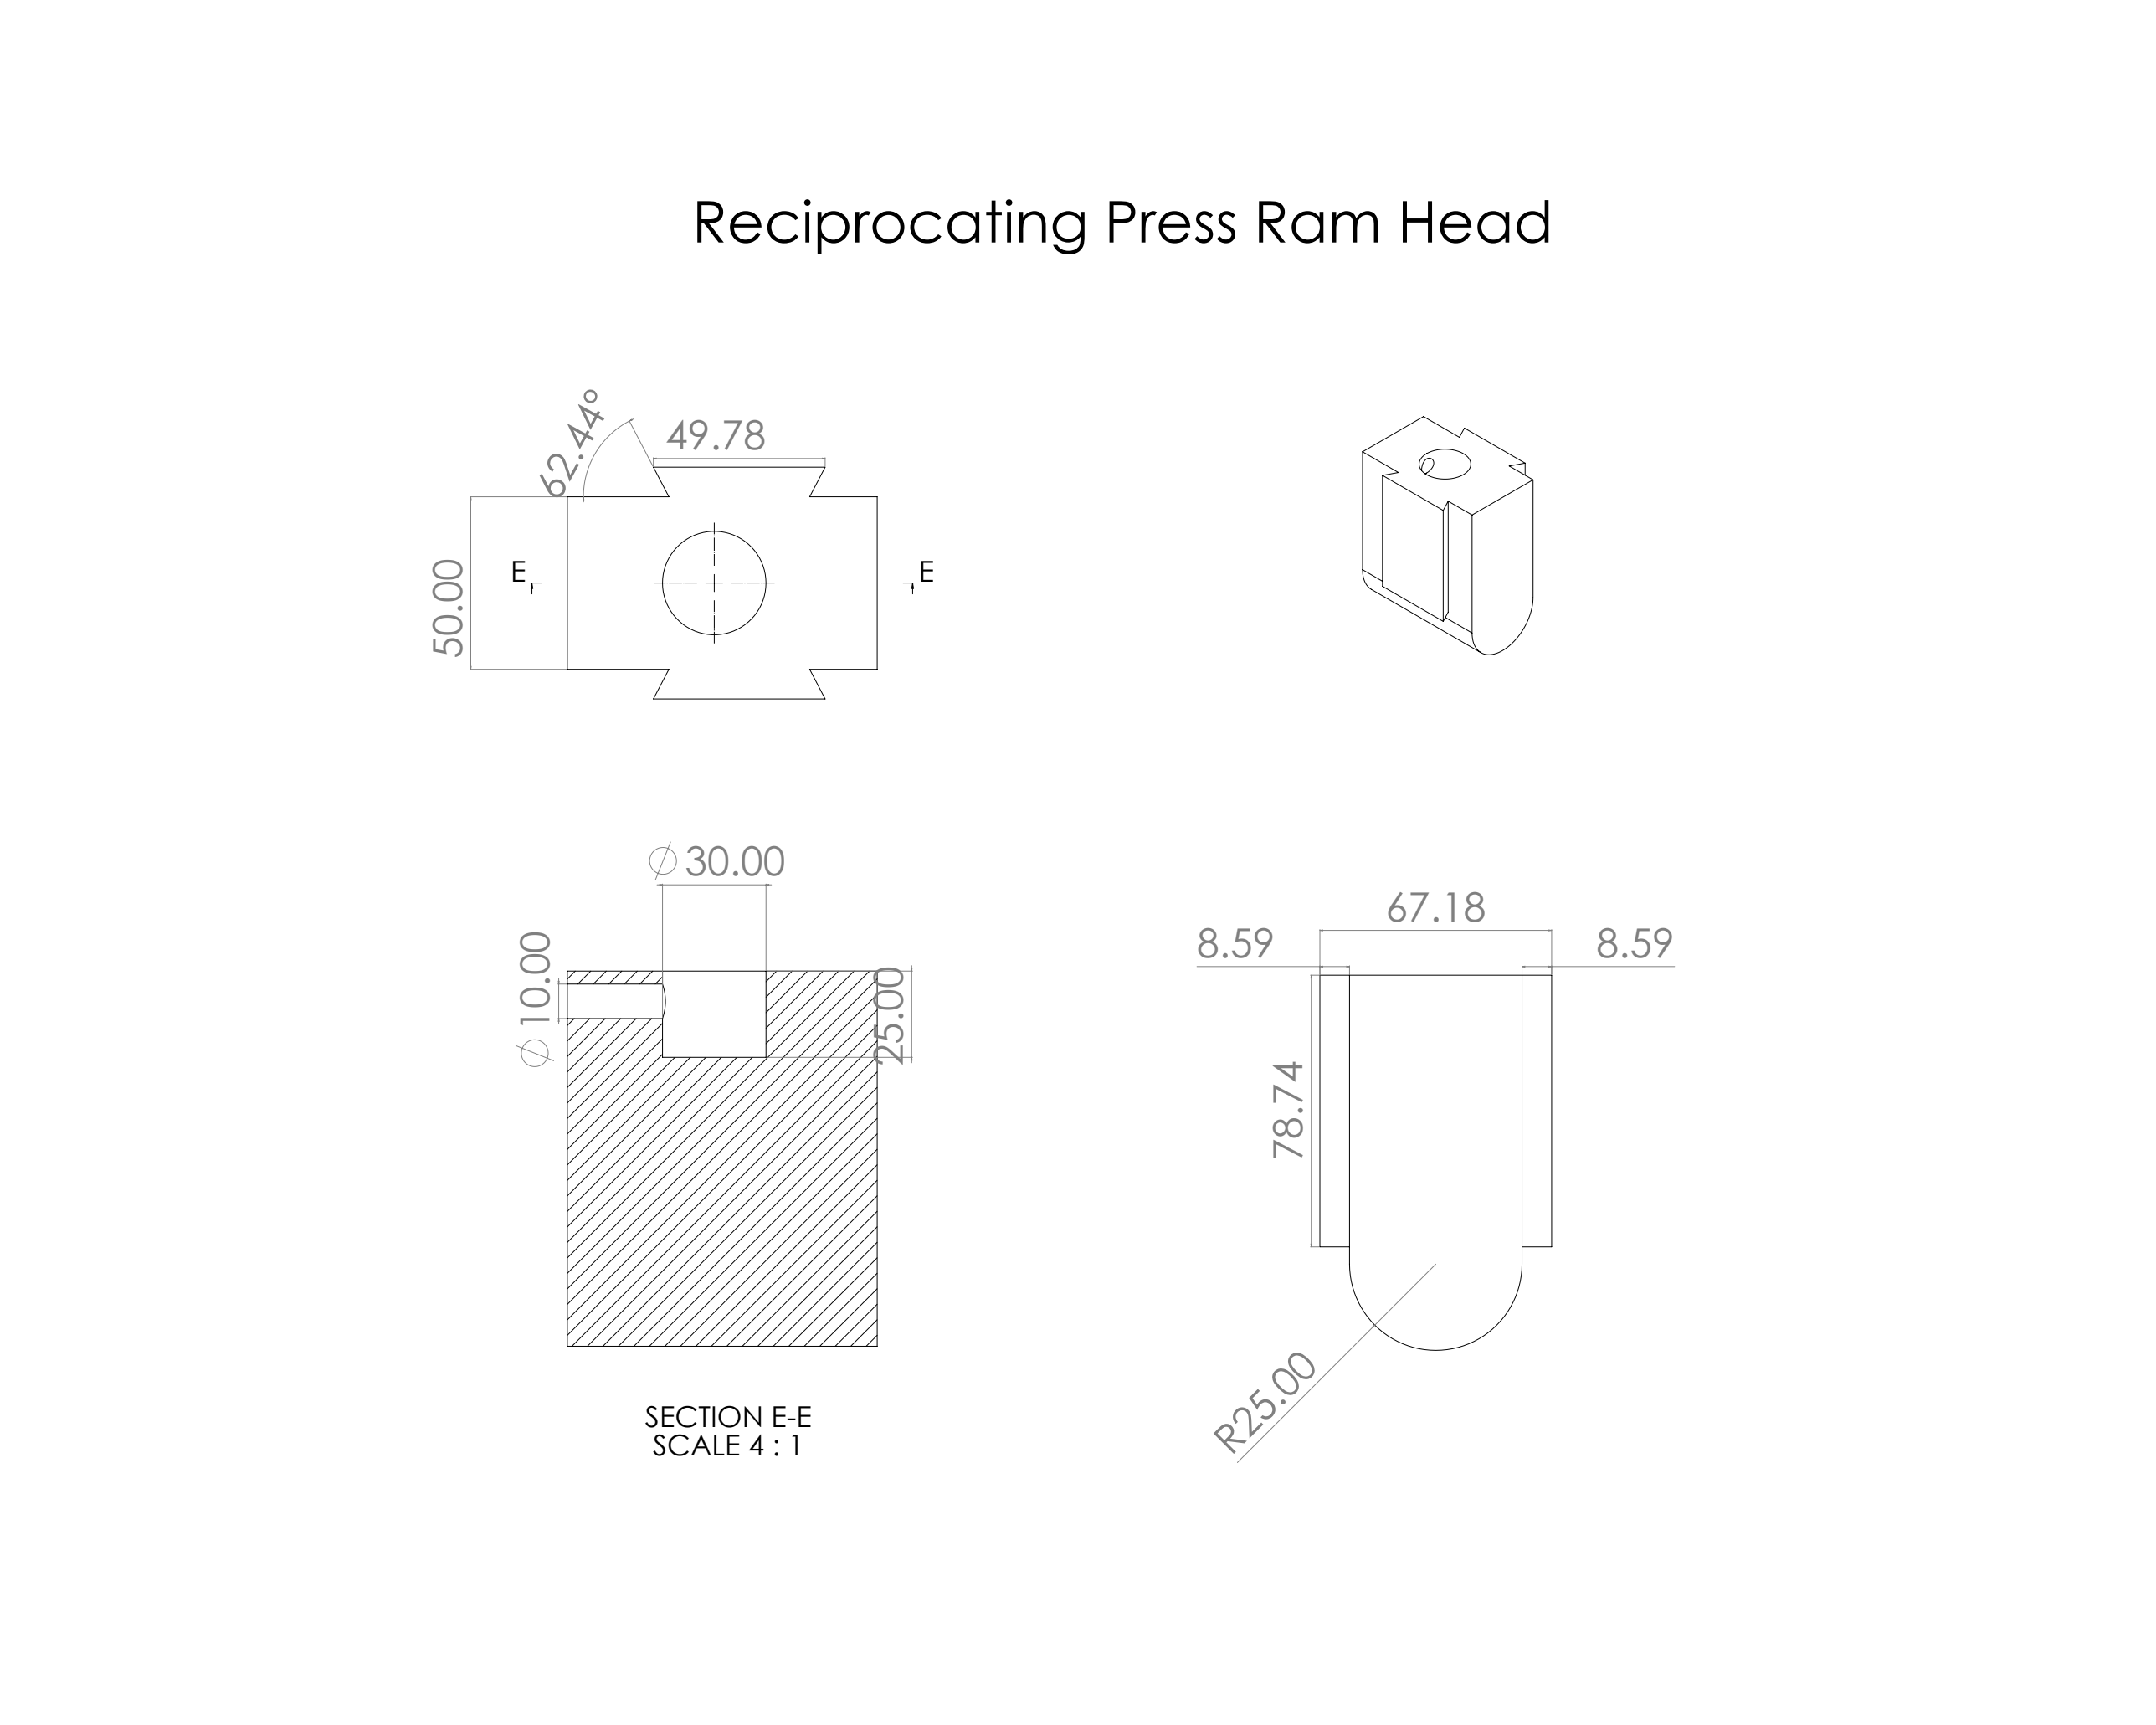
ISO-10303-21;
HEADER;
FILE_DESCRIPTION (('STEP AP214'),
    '1' );
FILE_NAME ('Reciprocating Press Ram Head.step',
    '2026-10-24T00:28:05',
    ( '' ),
    ( '' ),
    'SwSTEP 2.0',
    'SolidWorks 2025',
    '' );
FILE_SCHEMA (( 'AUTOMOTIVE_DESIGN' ));
ENDSEC;

DATA;
#14=CARTESIAN_POINT ( 'NONE',  ( -43.04716123355245827, 207.6569251493015429, -4.334626618252813479 ) ) ;
#38=EDGE_CURVE ( 'NONE', #12347, #13852, #5030, .T. ) ;
#51=CIRCLE ( 'NONE', #12122, 25.00000000000000711 ) ;
#74=VERTEX_POINT ( 'NONE', #5769 ) ;
#92=CARTESIAN_POINT ( 'NONE',  ( 3.458603197740078627, 135.1716627696692683, -33.59072564020503648 ) ) ;
#250=EDGE_CURVE ( 'NONE', #13614, #661, #3833, .T. ) ;
#262=ORIENTED_EDGE ( 'NONE', *, *, #2754, .T. ) ;
#275=CARTESIAN_POINT ( 'NONE',  ( 18.55315245287936321, 326.0737056351150613, 0.000000000000000000 ) ) ;
#276=DIRECTION ( 'NONE',  ( 1.000000000000000000, 0.000000000000000000, 0.000000000000000000 ) ) ;
#303=DIRECTION ( 'NONE',  ( 0.000000000000000000, -1.000000000000000000, 0.000000000000000000 ) ) ;
#324=PRODUCT_DEFINITION ( 'UNKNOWN', '', #14550, #16365 ) ;
#333=AXIS2_PLACEMENT_3D ( 'NONE', #2652, #9240, #18099 ) ;
#342=ORIENTED_EDGE ( 'NONE', *, *, #2095, .T. ) ;
#346=PLANE ( 'NONE',  #8685 ) ;
#375=SHAPE_DEFINITION_REPRESENTATION ( #12875, #7793 ) ;
#412=DIRECTION ( 'NONE',  ( -1.000000000000000000, 0.000000000000000000, -0.000000000000000000 ) ) ;
#463=ADVANCED_FACE ( 'NONE', ( #4898 ), #18196, .F. ) ;
#483=DIRECTION ( 'NONE',  ( 0.000000000000000000, -1.000000000000000000, 0.000000000000000000 ) ) ;
#546=ORIENTED_EDGE ( 'NONE', *, *, #13520, .F. ) ;
#560=EDGE_CURVE ( 'NONE', #9549, #9782, #17331, .T. ) ;
#593=CARTESIAN_POINT ( 'NONE',  ( -42.91927816222971614, 203.5270276421415190, -4.734255112268845878 ) ) ;
#601=VECTOR ( 'NONE', #13140, 999.9999999999998863 ) ;
#613=VECTOR ( 'NONE', #276, 1000.000000000000000 ) ;
#616=DIRECTION ( 'NONE',  ( -1.191790137725560488E-16, 1.000000000000000000, -0.000000000000000000 ) ) ;
#661=VERTEX_POINT ( 'NONE', #1116 ) ;
#674=CARTESIAN_POINT ( 'NONE',  ( -1.025382690249029949, 326.0737056351150613, 25.00000000000000000 ) ) ;
#696=DIRECTION ( 'NONE',  ( 1.000000000000000000, 0.000000000000000000, 0.000000000000000000 ) ) ;
#777=EDGE_CURVE ( 'NONE', #1912, #13157, #11419, .T. ) ;
#808=CARTESIAN_POINT ( 'NONE',  ( 0.000000000000000000, 0.000000000000000000, 0.000000000000000000 ) ) ;
#811=CARTESIAN_POINT ( 'NONE',  ( -43.67482055103364047, 200.1767183643995054, -0.6599055232175776720 ) ) ;
#849=AXIS2_PLACEMENT_3D ( 'NONE', #5042, #1929, #16634 ) ;
#854=DIRECTION ( 'NONE',  ( -1.000000000000000000, -0.000000000000000000, -0.000000000000000000 ) ) ;
#866=CARTESIAN_POINT ( 'NONE',  ( -1.025382690249028173, 213.9102039777116602, -25.00000000000000000 ) ) ;
#873=ORIENTED_EDGE ( 'NONE', *, *, #38, .F. ) ;
#897=ORIENTED_EDGE ( 'NONE', *, *, #15663, .F. ) ;
#937=FACE_OUTER_BOUND ( 'NONE', #6121, .T. ) ;
#962=DIRECTION ( 'NONE',  ( 0.000000000000000000, 0.000000000000000000, 1.000000000000000000 ) ) ;
#1045=CARTESIAN_POINT ( 'NONE',  ( -31.26501780185373391, 205.1437886375728965, 0.000000000000000000 ) ) ;
#1104=EDGE_CURVE ( 'NONE', #13157, #1912, #14909, .T. ) ;
#1113=AXIS2_PLACEMENT_3D ( 'NONE', #20332, #2170, #13424 ) ;
#1116=CARTESIAN_POINT ( 'NONE',  ( 3.458603197740078627, 213.9102039777116602, -33.59072564020503648 ) ) ;
#1153=FACE_OUTER_BOUND ( 'NONE', #10681, .T. ) ;
#1176=EDGE_CURVE ( 'NONE', #7385, #13157, #2466, .T. ) ;
#1212=ORIENTED_EDGE ( 'NONE', *, *, #6430, .T. ) ;
#1228=LINE ( 'NONE', #14432, #10712 ) ;
#1281=AXIS2_PLACEMENT_3D ( 'NONE', #20836, #19309, #9358 ) ;
#1284=EDGE_CURVE ( 'NONE', #6399, #21098, #51, .T. ) ;
#1288=ORIENTED_EDGE ( 'NONE', *, *, #5130, .F. ) ;
#1300=B_SPLINE_CURVE_WITH_KNOTS ( 'NONE', 3,
 ( #11564, #18152, #4544, #3349, #1735, #3030, #2927, #6576, #14505, #8308, #6261, #13199, #9507, #9614, #16231, #12766, #7875, #6152, #21296, #12873 ),
 .UNSPECIFIED., .F., .F.,
 ( 4, 2, 2, 2, 2, 2, 2, 2, 2, 4 ),
 ( 2.332952144782239016E-18, 0.0009844208871748760543, 0.001968841774349749506, 0.002953262661524623609, 0.003937683548699497278, 0.004922104435874371381, 0.005906525323049245484, 0.006398735766636720265, 0.006890946210224195914, 0.007875367097399143743 ),
 .UNSPECIFIED. ) ;
#1317=CARTESIAN_POINT ( 'NONE',  ( -43.15102588740141698, 208.1950015687324651, -3.974285180378252402 ) ) ;
#1370=ORIENTED_EDGE ( 'NONE', *, *, #11144, .T. ) ;
#1410=VECTOR ( 'NONE', #483, 1000.000000000000000 ) ;
#1419=CARTESIAN_POINT ( 'NONE',  ( -43.47609127650945737, 209.4774105891669933, -2.515022083182098189 ) ) ;
#1471=VERTEX_POINT ( 'NONE', #17701 ) ;
#1530=VECTOR ( 'NONE', #9051, 1000.000000000000000 ) ;
#1547=EDGE_LOOP ( 'NONE', ( #12729, #14512, #20221, #4392 ) ) ;
#1572=CARTESIAN_POINT ( 'NONE',  ( -43.15150032496258348, 208.1972798037766950, 3.972578417695639352 ) ) ;
#1670=DIRECTION ( 'NONE',  ( 0.8865057725575725689, 0.000000000000000000, 0.4627175328665443232 ) ) ;
#1703=DIRECTION ( 'NONE',  ( -1.000000000000000000, 0.000000000000000000, 0.000000000000000000 ) ) ;
#1713=CARTESIAN_POINT ( 'NONE',  ( -13.68588794268869790, 213.9102039777116602, 1.836970198721029589E-15 ) ) ;
#1731=CARTESIAN_POINT ( 'NONE',  ( -71.26501780185373036, 213.9102039777116602, 0.000000000000000000 ) ) ;
#1735=CARTESIAN_POINT ( 'NONE',  ( -43.60108677734861260, 200.4027425691367057, 1.621665263882683838 ) ) ;
#1762=CLOSED_SHELL ( 'NONE', ( #4254, #7700, #10763, #5705, #463, #10790, #10403, #16061, #9033, #19364, #19712, #8820, #7218, #3065, #7846, #20538, #4593, #3084, #19659 ) ) ;
#1775=VECTOR ( 'NONE', #9135, 1000.000000000000000 ) ;
#1776=AXIS2_PLACEMENT_3D ( 'NONE', #17630, #12444, #5836 ) ;
#1798=CARTESIAN_POINT ( 'NONE',  ( -43.47642916300955562, 209.4785612017895176, 2.513052019990858366 ) ) ;
#1846=CARTESIAN_POINT ( 'NONE',  ( 1.336753550880579347E-14, 213.9102039777116602, 25.00000000000000000 ) ) ;
#1896=CARTESIAN_POINT ( 'NONE',  ( 18.55315245287936321, 326.0737056351150613, 25.00000000000000000 ) ) ;
#1906=CARTESIAN_POINT ( 'NONE',  ( -43.68320130047528238, 210.1357463702879613, 0.3279153920022773727 ) ) ;
#1912=VERTEX_POINT ( 'NONE', #6308 ) ;
#1929=DIRECTION ( 'NONE',  ( -1.191790137725560488E-16, 1.000000000000000000, 0.000000000000000000 ) ) ;
#2094=VECTOR ( 'NONE', #11631, 1000.000000000000114 ) ;
#2095=EDGE_CURVE ( 'NONE', #11573, #6399, #18201, .T. ) ;
#2106=CARTESIAN_POINT ( 'NONE',  ( -43.31864445205426506, 201.3798797254112571, -3.307266650052995249 ) ) ;
#2121=VERTEX_POINT ( 'NONE', #8355 ) ;
#2170=DIRECTION ( 'NONE',  ( -1.000000000000000000, -0.000000000000000000, -0.000000000000000000 ) ) ;
#2193=CARTESIAN_POINT ( 'NONE',  ( -43.68588794268869435, 188.9102039777116602, 0.000000000000000000 ) ) ;
#2208=CARTESIAN_POINT ( 'NONE',  ( -43.37470026482863972, 201.1699573972600774, -3.051950158715578176 ) ) ;
#2235=PLANE ( 'NONE',  #7704 ) ;
#2269=ORIENTED_EDGE ( 'NONE', *, *, #15543, .T. ) ;
#2275=DIRECTION ( 'NONE',  ( 0.000000000000000000, 0.000000000000000000, -1.000000000000000000 ) ) ;
#2326=EDGE_LOOP ( 'NONE', ( #21282, #8318, #9603, #19499 ) ) ;
#2355=ORIENTED_EDGE ( 'NONE', *, *, #18512, .F. ) ;
#2419=DIRECTION ( 'NONE',  ( 0.000000000000000000, 0.000000000000000000, 1.000000000000000000 ) ) ;
#2422=DIRECTION ( 'NONE',  ( 0.4627175328665443232, 5.514621922230504147E-17, 0.8865057725575725689 ) ) ;
#2466=LINE ( 'NONE', #17179, #15585 ) ;
#2470=CARTESIAN_POINT ( 'NONE',  ( 1.336753550880579347E-14, 213.9102039777116602, -25.00000000000000000 ) ) ;
#2514=CARTESIAN_POINT ( 'NONE',  ( -46.31968306282883674, 326.0737056351150613, -33.59072564020502938 ) ) ;
#2554=LINE ( 'NONE', #8817, #1775 ) ;
#2611=EDGE_CURVE ( 'NONE', #18039, #6038, #13957, .T. ) ;
#2652=CARTESIAN_POINT ( 'NONE',  ( 0.000000000000000000, 326.0737056351150613, -33.59072564020503648 ) ) ;
#2754=EDGE_CURVE ( 'NONE', #10000, #13614, #15997, .T. ) ;
#2791=VECTOR ( 'NONE', #17043, 999.9999999999998863 ) ;
#2810=LINE ( 'NONE', #19027, #18368 ) ;
#2818=CARTESIAN_POINT ( 'NONE',  ( -71.26501780185373036, 135.1716627696692683, -25.00000000000000000 ) ) ;
#2841=DIRECTION ( 'NONE',  ( 1.191790137725560488E-16, -1.000000000000000000, 0.000000000000000000 ) ) ;
#2860=FACE_OUTER_BOUND ( 'NONE', #2326, .T. ) ;
#2875=DIRECTION ( 'NONE',  ( -1.000000000000000000, 0.000000000000000000, 0.000000000000000000 ) ) ;
#2885=EDGE_LOOP ( 'NONE', ( #4892, #17666 ) ) ;
#2927=CARTESIAN_POINT ( 'NONE',  ( -43.47648769733579854, 200.8087914445877971, 2.512805286998617049 ) ) ;
#2965=DIRECTION ( 'NONE',  ( -0.8865057725575725689, 0.000000000000000000, 0.4627175328665443232 ) ) ;
#2978=FACE_OUTER_BOUND ( 'NONE', #14370, .T. ) ;
#2988=ORIENTED_EDGE ( 'NONE', *, *, #21108, .T. ) ;
#3004=DIRECTION ( 'NONE',  ( 0.000000000000000000, 0.000000000000000000, 1.000000000000000000 ) ) ;
#3030=CARTESIAN_POINT ( 'NONE',  ( -43.52287249567941529, 200.6548609068916278, 2.226397062484288814 ) ) ;
#3065=ADVANCED_FACE ( 'NONE', ( #16524, #8276 ), #13386, .T. ) ;
#3066=AXIS2_PLACEMENT_3D ( 'NONE', #16187, #11087, #4703 ) ;
#3084=ADVANCED_FACE ( 'NONE', ( #13280 ), #3533, .T. ) ;
#3104=CARTESIAN_POINT ( 'NONE',  ( -28.68588794268869435, 188.9102039777116602, 0.000000000000000000 ) ) ;
#3152=VECTOR ( 'NONE', #5219, 1000.000000000000000 ) ;
#3194=CARTESIAN_POINT ( 'NONE',  ( -43.04742826731176564, 207.6584868706943041, 4.333760535973598671 ) ) ;
#3226=VECTOR ( 'NONE', #10704, 1000.000000000000000 ) ;
#3249=ORIENTED_EDGE ( 'NONE', *, *, #10862, .T. ) ;
#3255=CARTESIAN_POINT ( 'NONE',  ( -43.31915179403467420, 208.9097650327693430, -3.305147470758842410 ) ) ;
#3297=DIRECTION ( 'NONE',  ( 0.8865057725575725689, 0.000000000000000000, 0.4627175328665443232 ) ) ;
#3308=ORIENTED_EDGE ( 'NONE', *, *, #21108, .F. ) ;
#3314=ORIENTED_EDGE ( 'NONE', *, *, #18512, .T. ) ;
#3321=DIRECTION ( 'NONE',  ( 0.000000000000000000, -0.000000000000000000, -1.000000000000000000 ) ) ;
#3332=VECTOR ( 'NONE', #8114, 1000.000000000000000 ) ;
#3349=CARTESIAN_POINT ( 'NONE',  ( -43.63268616469407846, 200.3053519615658615, 1.302651870180923321 ) ) ;
#3359=VERTEX_POINT ( 'NONE', #2193 ) ;
#3397=DIRECTION ( 'NONE',  ( 0.000000000000000000, -1.000000000000000000, 0.000000000000000000 ) ) ;
#3415=ORIENTED_EDGE ( 'NONE', *, *, #8284, .T. ) ;
#3448=CARTESIAN_POINT ( 'NONE',  ( -41.83569717483972994, 135.1716627696692683, -24.99999999999998934 ) ) ;
#3488=( GEOMETRIC_REPRESENTATION_CONTEXT ( 3 ) GLOBAL_UNCERTAINTY_ASSIGNED_CONTEXT ( ( #13089 ) ) GLOBAL_UNIT_ASSIGNED_CONTEXT ( ( #13667, #8565, #20256 ) ) REPRESENTATION_CONTEXT ( 'NONE', 'WORKASPACE' ) );
#3507=CARTESIAN_POINT ( 'NONE',  ( -22.62331590640576096, 213.9102039777116602, -11.80838889663596447 ) ) ;
#3524=AXIS2_PLACEMENT_3D ( 'NONE', #11422, #7749, #3004 ) ;
#3533=PLANE ( 'NONE',  #849 ) ;
#3542=EDGE_CURVE ( 'NONE', #16754, #11704, #13661, .T. ) ;
#3567=VERTEX_POINT ( 'NONE', #5738 ) ;
#3679=ORIENTED_EDGE ( 'NONE', *, *, #2611, .T. ) ;
#3786=EDGE_CURVE ( 'NONE', #15417, #3359, #12531, .T. ) ;
#3794=ORIENTED_EDGE ( 'NONE', *, *, #5782, .T. ) ;
#3830=DIRECTION ( 'NONE',  ( -0.8865057725575725689, 0.000000000000000000, 0.4627175328665443232 ) ) ;
#3833=LINE ( 'NONE', #7069, #2791 ) ;
#3840=VECTOR ( 'NONE', #2422, 999.9999999999998863 ) ;
#3876=CARTESIAN_POINT ( 'NONE',  ( -22.62331590640576451, 135.1716627696692683, -11.80838889663595914 ) ) ;
#3922=EDGE_CURVE ( 'NONE', #14679, #13370, #6472, .T. ) ;
#3937=CARTESIAN_POINT ( 'NONE',  ( -43.68588794268869435, 200.1437886375728965, 2.403080215999224424E-15 ) ) ;
#3952=DIRECTION ( 'NONE',  ( -1.000000000000000000, -1.191790137725560488E-16, 0.000000000000000000 ) ) ;
#3982=ORIENTED_EDGE ( 'NONE', *, *, #15019, .F. ) ;
#3983=ORIENTED_EDGE ( 'NONE', *, *, #17042, .T. ) ;
#4031=CARTESIAN_POINT ( 'NONE',  ( -22.62331590640576096, 213.9102039777116602, 11.80838889663596447 ) ) ;
#4043=FACE_OUTER_BOUND ( 'NONE', #8124, .T. ) ;
#4177=EDGE_LOOP ( 'NONE', ( #3308, #13446, #6905, #1212 ) ) ;
#4245=AXIS2_PLACEMENT_3D ( 'NONE', #13600, #303, #3321 ) ;
#4254=ADVANCED_FACE ( 'NONE', ( #6341 ), #7319, .F. ) ;
#4312=DIRECTION ( 'NONE',  ( -0.4627175328665442677, 0.000000000000000000, 0.8865057725575725689 ) ) ;
#4315=CARTESIAN_POINT ( 'NONE',  ( -1.025382690249029949, 213.9102039777116602, 25.00000000000000000 ) ) ;
#4335=EDGE_CURVE ( 'NONE', #6728, #10701, #7955, .T. ) ;
#4342=ORIENTED_EDGE ( 'NONE', *, *, #777, .T. ) ;
#4379=DIRECTION ( 'NONE',  ( 0.000000000000000000, -1.000000000000000000, 0.000000000000000000 ) ) ;
#4387=AXIS2_PLACEMENT_3D ( 'NONE', #9664, #8472, #8251 ) ;
#4392=ORIENTED_EDGE ( 'NONE', *, *, #1284, .F. ) ;
#4443=ORIENTED_EDGE ( 'NONE', *, *, #4335, .T. ) ;
#4447=PLANE ( 'NONE',  #8269 ) ;
#4449=DIRECTION ( 'NONE',  ( 0.000000000000000000, 0.000000000000000000, 1.000000000000000000 ) ) ;
#4452=FACE_BOUND ( 'NONE', #15353, .T. ) ;
#4489=LINE ( 'NONE', #12925, #9062 ) ;
#4544=CARTESIAN_POINT ( 'NONE',  ( -43.67481775055303928, 200.1767262095909246, 0.6600471188826699809 ) ) ;
#4553=CARTESIAN_POINT ( 'NONE',  ( -42.91697296918459159, 206.7606908932681051, -4.742769269235594720 ) ) ;
#4593=ADVANCED_FACE ( 'NONE', ( #1153 ), #16179, .F. ) ;
#4613=CARTESIAN_POINT ( 'NONE',  ( -13.68588794268869435, 188.9102039777116602, 1.836970198721029983E-15 ) ) ;
#4646=LINE ( 'NONE', #16443, #16857 ) ;
#4663=DIRECTION ( 'NONE',  ( 1.000000000000000000, 1.191790137725560488E-16, 0.000000000000000000 ) ) ;
#4691=CARTESIAN_POINT ( 'NONE',  ( -71.26501780185373036, 130.1716627696692683, 25.00000000000000000 ) ) ;
#4703=DIRECTION ( 'NONE',  ( -1.000000000000000000, 0.000000000000000000, 0.000000000000000000 ) ) ;
#4757=CARTESIAN_POINT ( 'NONE',  ( -42.88446638378037079, 206.4484180351192322, -4.837872587287148640 ) ) ;
#4764=CARTESIAN_POINT ( 'NONE',  ( -28.68588794268869790, 213.9102039777116602, 0.000000000000000000 ) ) ;
#4773=CARTESIAN_POINT ( 'NONE',  ( -42.82802356641964536, 205.1437886375728965, -5.000000000000001776 ) ) ;
#4892=ORIENTED_EDGE ( 'NONE', *, *, #1104, .F. ) ;
#4898=FACE_OUTER_BOUND ( 'NONE', #12108, .T. ) ;
#4920=VERTEX_POINT ( 'NONE', #20370 ) ;
#4926=EDGE_CURVE ( 'NONE', #13370, #10360, #12699, .T. ) ;
#4933=DIRECTION ( 'NONE',  ( -1.191790137725560488E-16, 1.000000000000000000, 0.000000000000000000 ) ) ;
#4946=VECTOR ( 'NONE', #13315, 1000.000000000000000 ) ;
#4962=LINE ( 'NONE', #2818, #8189 ) ;
#4973=ORIENTED_EDGE ( 'NONE', *, *, #2754, .F. ) ;
#5019=CARTESIAN_POINT ( 'NONE',  ( -43.37443857369948574, 209.1166545091122657, 3.053198389463522844 ) ) ;
#5021=CARTESIAN_POINT ( 'NONE',  ( 1.336753550880579347E-14, 213.9102039777116602, 33.59072564020503648 ) ) ;
#5030=LINE ( 'NONE', #18331, #2094 ) ;
#5033=ORIENTED_EDGE ( 'NONE', *, *, #4335, .F. ) ;
#5042=CARTESIAN_POINT ( 'NONE',  ( -28.68588794268869435, 188.9102039777116602, 0.000000000000000000 ) ) ;
#5077=EDGE_CURVE ( 'NONE', #9549, #20916, #15731, .T. ) ;
#5120=FACE_OUTER_BOUND ( 'NONE', #14147, .T. ) ;
#5130=EDGE_CURVE ( 'NONE', #1471, #2121, #1228, .T. ) ;
#5135=AXIS2_PLACEMENT_3D ( 'NONE', #4764, #2841, #4663 ) ;
#5215=ORIENTED_EDGE ( 'NONE', *, *, #250, .T. ) ;
#5219=DIRECTION ( 'NONE',  ( 0.000000000000000000, -1.000000000000000000, 0.000000000000000000 ) ) ;
#5265=ORIENTED_EDGE ( 'NONE', *, *, #5077, .T. ) ;
#5460=CARTESIAN_POINT ( 'NONE',  ( 1.631480618821192334E-14, 213.9102039777116602, -24.99999999999999645 ) ) ;
#5464=LINE ( 'NONE', #1731, #10962 ) ;
#5507=ORIENTED_EDGE ( 'NONE', *, *, #20586, .F. ) ;
#5529=DIRECTION ( 'NONE',  ( -0.4627175328665442677, 0.000000000000000000, -0.8865057725575725689 ) ) ;
#5616=ORIENTED_EDGE ( 'NONE', *, *, #5775, .F. ) ;
#5629=ORIENTED_EDGE ( 'NONE', *, *, #2095, .F. ) ;
#5634=LINE ( 'NONE', #17220, #3226 ) ;
#5675=DIRECTION ( 'NONE',  ( 1.000000000000000000, 1.191790137725560488E-16, 1.178908271762451515E-16 ) ) ;
#5677=CARTESIAN_POINT ( 'NONE',  ( -41.83569717483972994, 213.9102039777116602, -25.00000000000000000 ) ) ;
#5705=ADVANCED_FACE ( 'NONE', ( #10914 ), #17526, .T. ) ;
#5738=CARTESIAN_POINT ( 'NONE',  ( -43.68588794268869435, 213.9102039777116602, 0.000000000000000000 ) ) ;
#5769=CARTESIAN_POINT ( 'NONE',  ( -71.26501780185373036, 213.9102039777116602, 25.00000000000000355 ) ) ;
#5775=EDGE_CURVE ( 'NONE', #18006, #3567, #13504, .T. ) ;
#5782=EDGE_CURVE ( 'NONE', #10000, #11573, #19357, .T. ) ;
#5836=DIRECTION ( 'NONE',  ( -1.000000000000000000, 0.000000000000000000, 0.000000000000000000 ) ) ;
#5848=ORIENTED_EDGE ( 'NONE', *, *, #1176, .T. ) ;
#5866=CARTESIAN_POINT ( 'NONE',  ( -42.88696169552118675, 203.8418613323790396, -4.830328443944832628 ) ) ;
#5969=( NAMED_UNIT ( * ) PLANE_ANGLE_UNIT ( ) SI_UNIT ( $, .RADIAN. ) );
#6018=ORIENTED_EDGE ( 'NONE', *, *, #12630, .T. ) ;
#6038=VERTEX_POINT ( 'NONE', #11054 ) ;
#6055=ORIENTED_EDGE ( 'NONE', *, *, #560, .F. ) ;
#6121=EDGE_LOOP ( 'NONE', ( #15052, #21157, #12224, #6055 ) ) ;
#6149=CARTESIAN_POINT ( 'NONE',  ( 18.55315245287936321, 213.9102039777116602, -25.00000000000000000 ) ) ;
#6152=CARTESIAN_POINT ( 'NONE',  ( -42.83951137863823533, 204.4886979175576016, 4.967857365464206865 ) ) ;
#6261=CARTESIAN_POINT ( 'NONE',  ( -43.15146482487497792, 202.0901544311013538, 3.972812079771462113 ) ) ;
#6301=EDGE_CURVE ( 'NONE', #74, #4920, #5634, .T. ) ;
#6308=CARTESIAN_POINT ( 'NONE',  ( -71.26501780185373036, 205.1437886375728965, -5.000000000000001776 ) ) ;
#6341=FACE_OUTER_BOUND ( 'NONE', #20011, .T. ) ;
#6375=CARTESIAN_POINT ( 'NONE',  ( -43.63240530816146645, 209.9813655751484305, -1.306613905557860500 ) ) ;
#6399=VERTEX_POINT ( 'NONE', #16452 ) ;
#6430=EDGE_CURVE ( 'NONE', #6038, #16754, #8207, .T. ) ;
#6445=EDGE_CURVE ( 'NONE', #2121, #4920, #17049, .T. ) ;
#6472=B_SPLINE_CURVE_WITH_KNOTS ( 'NONE', 3,
 ( #16134, #21099, #16243, #6375, #11247, #17845, #1419, #14837, #3255, #6480, #1317, #14, #19576, #4553, #4757, #6588, #11574, #7888 ),
 .UNSPECIFIED., .F., .F.,
 ( 4, 2, 2, 2, 2, 2, 2, 2, 4 ),
 ( 0.01574578602456870244, 0.01672957298347709995, 0.01771335994238549399, 0.01869714690129389151, 0.01968093386020228555, 0.02066472081911068306, 0.02164850777801907711, 0.02263229473692747462, 0.02361608169583586866 ),
 .UNSPECIFIED. ) ;
#6480=CARTESIAN_POINT ( 'NONE',  ( -43.20717515250593266, 208.4480206960199382, -3.766779594902115225 ) ) ;
#6497=LINE ( 'NONE', #14958, #11620 ) ;
#6512=DIRECTION ( 'NONE',  ( 0.4627175328665442677, 0.000000000000000000, -0.8865057725575724579 ) ) ;
#6522=LINE ( 'NONE', #3507, #601 ) ;
#6537=ORIENTED_EDGE ( 'NONE', *, *, #6301, .T. ) ;
#6555=LINE ( 'NONE', #13175, #21295 ) ;
#6576=CARTESIAN_POINT ( 'NONE',  ( -43.37414277151795261, 201.1719893629813498, 3.054701555947804792 ) ) ;
#6588=CARTESIAN_POINT ( 'NONE',  ( -42.83993802355417557, 205.8067832142903910, -4.966639429937480088 ) ) ;
#6599=DIRECTION ( 'NONE',  ( -1.191790137725560488E-16, 1.000000000000000000, -0.000000000000000000 ) ) ;
#6634=CARTESIAN_POINT ( 'NONE',  ( -42.88454851406326185, 206.4494888775581103, 4.837634058829628714 ) ) ;
#6726=ORIENTED_EDGE ( 'NONE', *, *, #17290, .T. ) ;
#6728=VERTEX_POINT ( 'NONE', #4315 ) ;
#6745=CARTESIAN_POINT ( 'NONE',  ( -42.82802356641963826, 205.4725094246604442, 5.000000000000000888 ) ) ;
#6755=ORIENTED_EDGE ( 'NONE', *, *, #15009, .T. ) ;
#6783=ORIENTED_EDGE ( 'NONE', *, *, #12630, .F. ) ;
#6835=LINE ( 'NONE', #20042, #3152 ) ;
#6850=CARTESIAN_POINT ( 'NONE',  ( -43.68588794268869435, 210.1437886375728965, -2.161864096862809871E-19 ) ) ;
#6903=EDGE_LOOP ( 'NONE', ( #8636, #14114, #13505, #19365, #10872, #20519, #6907 ) ) ;
#6905=ORIENTED_EDGE ( 'NONE', *, *, #15663, .T. ) ;
#6907=ORIENTED_EDGE ( 'NONE', *, *, #15009, .F. ) ;
#6963=ORIENTED_EDGE ( 'NONE', *, *, #15543, .F. ) ;
#6967=ORIENTED_EDGE ( 'NONE', *, *, #15708, .T. ) ;
#7012=EDGE_LOOP ( 'NONE', ( #17895, #9415, #8615, #20147 ) ) ;
#7058=CARTESIAN_POINT ( 'NONE',  ( -42.83955070047272073, 204.4880047785818533, -4.967744786903342202 ) ) ;
#7069=CARTESIAN_POINT ( 'NONE',  ( -11.06088464903279878, 213.9102039777116602, -5.773301668816275267 ) ) ;
#7080=LINE ( 'NONE', #7184, #9238 ) ;
#7160=CARTESIAN_POINT ( 'NONE',  ( -43.52298375438361688, 200.6544955639567434, -2.225641045960684128 ) ) ;
#7180=CARTESIAN_POINT ( 'NONE',  ( -43.68588794268869435, 188.9102039777116602, 0.000000000000000000 ) ) ;
#7184=CARTESIAN_POINT ( 'NONE',  ( -46.31968306282883674, 326.0737056351150613, 33.59072564020503648 ) ) ;
#7195=ORIENTED_EDGE ( 'NONE', *, *, #3786, .T. ) ;
#7201=ORIENTED_EDGE ( 'NONE', *, *, #1104, .T. ) ;
#7218=ADVANCED_FACE ( 'NONE', ( #2860 ), #17667, .T. ) ;
#7286=VERTEX_POINT ( 'NONE', #11058 ) ;
#7319=CYLINDRICAL_SURFACE ( 'NONE', #3524, 5.000000000000001776 ) ;
#7336=ORIENTED_EDGE ( 'NONE', *, *, #3542, .T. ) ;
#7350=ORIENTED_EDGE ( 'NONE', *, *, #7856, .F. ) ;
#7385=VERTEX_POINT ( 'NONE', #12073 ) ;
#7461=ORIENTED_EDGE ( 'NONE', *, *, #16181, .F. ) ;
#7544=CIRCLE ( 'NONE', #8583, 15.00000000000000355 ) ;
#7700=ADVANCED_FACE ( 'NONE', ( #19524 ), #13149, .F. ) ;
#7701=AXIS2_PLACEMENT_3D ( 'NONE', #20118, #18058, #11680 ) ;
#7704=AXIS2_PLACEMENT_3D ( 'NONE', #11854, #18551, #412 ) ;
#7749=DIRECTION ( 'NONE',  ( -1.000000000000000000, -0.000000000000000000, -0.000000000000000000 ) ) ;
#7774=CARTESIAN_POINT ( 'NONE',  ( -41.83569717483972994, 326.0737056351150613, 24.99999999999998934 ) ) ;
#7793=SHAPE_REPRESENTATION ( 'Reciprocating Press Ram Head', ( #12794 ), #14195 ) ;
#7795=LINE ( 'NONE', #20478, #18265 ) ;
#7846=ADVANCED_FACE ( 'NONE', ( #4452, #16461 ), #19689, .F. ) ;
#7856=EDGE_CURVE ( 'NONE', #11704, #18039, #8000, .T. ) ;
#7875=CARTESIAN_POINT ( 'NONE',  ( -42.87299489053027912, 204.0036020648173292, 4.871053504435129078 ) ) ;
#7888=CARTESIAN_POINT ( 'NONE',  ( -42.82802356641964536, 205.1437886375728965, -5.000000000000001776 ) ) ;
#7890=LINE ( 'NONE', #20279, #13820 ) ;
#7899=ADVANCED_BREP_SHAPE_REPRESENTATION ( '', ( #12161, #12794 ), #14195 ) ;
#7955=LINE ( 'NONE', #21170, #17343 ) ;
#8000=LINE ( 'NONE', #17956, #20325 ) ;
#8006=CARTESIAN_POINT ( 'NONE',  ( 3.458603197740078627, 135.1716627696692683, 33.59072564020503648 ) ) ;
#8047=ORIENTED_EDGE ( 'NONE', *, *, #14360, .F. ) ;
#8114=DIRECTION ( 'NONE',  ( 0.000000000000000000, -1.000000000000000000, 0.000000000000000000 ) ) ;
#8124=EDGE_LOOP ( 'NONE', ( #2355, #4443, #2988, #7336 ) ) ;
#8151=ORIENTED_EDGE ( 'NONE', *, *, #15576, .T. ) ;
#8189=VECTOR ( 'NONE', #9402, 1000.000000000000000 ) ;
#8207=LINE ( 'NONE', #9938, #4946 ) ;
#8251=DIRECTION ( 'NONE',  ( -1.000000000000000000, 0.000000000000000000, -0.000000000000000000 ) ) ;
#8269=AXIS2_PLACEMENT_3D ( 'NONE', #11032, #3830, #10419 ) ;
#8274=DIRECTION ( 'NONE',  ( 1.000000000000000000, 1.191790137725560488E-16, -1.178908271762451515E-16 ) ) ;
#8276=FACE_OUTER_BOUND ( 'NONE', #7012, .T. ) ;
#8284=EDGE_CURVE ( 'NONE', #3359, #15417, #7544, .T. ) ;
#8308=CARTESIAN_POINT ( 'NONE',  ( -43.20715004130836689, 201.8397834041948613, 3.766744768033092328 ) ) ;
#8318=ORIENTED_EDGE ( 'NONE', *, *, #560, .T. ) ;
#8355=CARTESIAN_POINT ( 'NONE',  ( -71.26501780185373036, 130.1716627696692683, -25.00000000000000355 ) ) ;
#8389=CARTESIAN_POINT ( 'NONE',  ( -71.26501780185373036, 326.0737056351150613, 0.000000000000000000 ) ) ;
#8472=DIRECTION ( 'NONE',  ( 0.000000000000000000, 0.000000000000000000, -1.000000000000000000 ) ) ;
#8474=CARTESIAN_POINT ( 'NONE',  ( -43.67243589781770652, 210.1033101532991338, 0.6559853996653204344 ) ) ;
#8536=CYLINDRICAL_SURFACE ( 'NONE', #1113, 25.00000000000000711 ) ;
#8565=( NAMED_UNIT ( * ) PLANE_ANGLE_UNIT ( ) SI_UNIT ( $, .RADIAN. ) );
#8583=AXIS2_PLACEMENT_3D ( 'NONE', #3104, #4933, #1703 ) ;
#8615=ORIENTED_EDGE ( 'NONE', *, *, #6301, .F. ) ;
#8636=ORIENTED_EDGE ( 'NONE', *, *, #3786, .F. ) ;
#8685=AXIS2_PLACEMENT_3D ( 'NONE', #18488, #2275, #15374 ) ;
#8709=CARTESIAN_POINT ( 'NONE',  ( 1.631480618821192334E-14, 213.9102039777116602, 24.99999999999999645 ) ) ;
#8817=CARTESIAN_POINT ( 'NONE',  ( -31.26501780185373391, 205.1437886375728965, -5.000000000000001776 ) ) ;
#8820=ADVANCED_FACE ( 'NONE', ( #937 ), #17463, .T. ) ;
#8828=ORIENTED_EDGE ( 'NONE', *, *, #1176, .F. ) ;
#8860=CIRCLE ( 'NONE', #1281, 15.00000000000000000 ) ;
#8870=LINE ( 'NONE', #674, #11493 ) ;
#8918=FACE_OUTER_BOUND ( 'NONE', #11911, .T. ) ;
#8938=DIRECTION ( 'NONE',  ( -1.000000000000000000, 0.000000000000000000, 0.000000000000000000 ) ) ;
#8975=UNCERTAINTY_MEASURE_WITH_UNIT (LENGTH_MEASURE( 1.000000000000000082E-05 ), #15936, 'distance_accuracy_value', 'NONE');
#9033=ADVANCED_FACE ( 'NONE', ( #5120 ), #10192, .F. ) ;
#9043=CARTESIAN_POINT ( 'NONE',  ( 18.55315245287936321, 213.9102039777116602, 25.00000000000000000 ) ) ;
#9051=DIRECTION ( 'NONE',  ( -1.000000000000000000, -1.191790137725560488E-16, 0.000000000000000000 ) ) ;
#9062=VECTOR ( 'NONE', #4379, 1000.000000000000000 ) ;
#9109=CARTESIAN_POINT ( 'NONE',  ( -43.20748696942038691, 201.8382954020869420, -3.765466433758053011 ) ) ;
#9135=DIRECTION ( 'NONE',  ( -1.000000000000000000, -0.000000000000000000, -0.000000000000000000 ) ) ;
#9197=DIRECTION ( 'NONE',  ( -1.000000000000000000, 0.000000000000000000, 0.000000000000000000 ) ) ;
#9218=VECTOR ( 'NONE', #616, 1000.000000000000000 ) ;
#9238=VECTOR ( 'NONE', #13807, 1000.000000000000000 ) ;
#9240=DIRECTION ( 'NONE',  ( 0.000000000000000000, 0.000000000000000000, -1.000000000000000000 ) ) ;
#9297=CARTESIAN_POINT ( 'NONE',  ( 18.55315245287936321, 213.9102039777116602, 0.000000000000000000 ) ) ;
#9348=EDGE_CURVE ( 'NONE', #14679, #3567, #7795, .T. ) ;
#9358=DIRECTION ( 'NONE',  ( -1.000000000000000000, 0.000000000000000000, 0.000000000000000000 ) ) ;
#9395=ORIENTED_EDGE ( 'NONE', *, *, #11250, .T. ) ;
#9398=AXIS2_PLACEMENT_3D ( 'NONE', #10969, #11394, #2875 ) ;
#9402=DIRECTION ( 'NONE',  ( 1.000000000000000000, 0.000000000000000000, 0.000000000000000000 ) ) ;
#9415=ORIENTED_EDGE ( 'NONE', *, *, #6445, .T. ) ;
#9507=CARTESIAN_POINT ( 'NONE',  ( -42.99819559747531628, 202.9232509211816478, 4.491669896562675568 ) ) ;
#9512=ORIENTED_EDGE ( 'NONE', *, *, #20586, .T. ) ;
#9549=VERTEX_POINT ( 'NONE', #12897 ) ;
#9583=PRODUCT ( 'Reciprocating Press Ram Head', 'Reciprocating Press Ram Head', '', ( #18416 ) ) ;
#9603=ORIENTED_EDGE ( 'NONE', *, *, #10862, .F. ) ;
#9614=CARTESIAN_POINT ( 'NONE',  ( -42.93756312153262655, 203.3739285472156268, 4.679109617540635924 ) ) ;
#9664=CARTESIAN_POINT ( 'NONE',  ( 0.000000000000000000, 326.0737056351150613, 25.00000000000000000 ) ) ;
#9681=ORIENTED_EDGE ( 'NONE', *, *, #17363, .F. ) ;
#9735=DIRECTION ( 'NONE',  ( -1.000000000000000000, -0.000000000000000000, -0.000000000000000000 ) ) ;
#9782=VERTEX_POINT ( 'NONE', #16997 ) ;
#9861=CARTESIAN_POINT ( 'NONE',  ( -22.62331590640576451, 326.0737056351150613, -11.80838889663595914 ) ) ;
#9901=FACE_OUTER_BOUND ( 'NONE', #10791, .T. ) ;
#9938=CARTESIAN_POINT ( 'NONE',  ( 0.000000000000000000, 135.1716627696692683, 33.59072564020503648 ) ) ;
#9967=VECTOR ( 'NONE', #3397, 1000.000000000000000 ) ;
#9985=CARTESIAN_POINT ( 'NONE',  ( -42.99906419454241302, 207.3703986995724335, 4.488953568700488006 ) ) ;
#10000=VERTEX_POINT ( 'NONE', #6149 ) ;
#10095=CARTESIAN_POINT ( 'NONE',  ( -43.63240380007613339, 209.9813597091836641, 1.306460585600322188 ) ) ;
#10127=DIRECTION ( 'NONE',  ( 1.000000000000000000, 0.000000000000000000, 0.000000000000000000 ) ) ;
#10192=PLANE ( 'NONE',  #18959 ) ;
#10281=VERTEX_POINT ( 'NONE', #3448 ) ;
#10300=CARTESIAN_POINT ( 'NONE',  ( -43.04679578547634122, 202.6324317550694616, -4.335932898175371975 ) ) ;
#10340=CARTESIAN_POINT ( 'NONE',  ( 0.000000000000000000, 130.1716627696692683, -25.00000000000000000 ) ) ;
#10358=EDGE_LOOP ( 'NONE', ( #3415, #7195 ) ) ;
#10360=VERTEX_POINT ( 'NONE', #3937 ) ;
#10382=DIRECTION ( 'NONE',  ( 0.000000000000000000, -1.000000000000000000, 0.000000000000000000 ) ) ;
#10403=ADVANCED_FACE ( 'NONE', ( #4043 ), #4447, .F. ) ;
#10409=CARTESIAN_POINT ( 'NONE',  ( -42.93765923600280843, 203.3731313234725917, -4.678819197459183954 ) ) ;
#10419=DIRECTION ( 'NONE',  ( 0.4627175328665442677, 0.000000000000000000, 0.8865057725575724579 ) ) ;
#10452=VERTEX_POINT ( 'NONE', #16136 ) ;
#10463=EDGE_CURVE ( 'NONE', #661, #9549, #7890, .T. ) ;
#10479=VECTOR ( 'NONE', #4312, 1000.000000000000114 ) ;
#10545=B_SPLINE_CURVE_WITH_KNOTS ( 'NONE', 3,
 ( #11833, #6745, #17999, #6634, #18428, #9985, #3194, #1572, #14772, #11727, #5019, #1798, #13361, #18320, #10095, #16717, #8474, #1906, #15097, #6850 ),
 .UNSPECIFIED., .F., .F.,
 ( 4, 2, 2, 2, 2, 2, 2, 2, 2, 4 ),
 ( 0.007875367097399143743, 0.008859169463295337929, 0.009842971829191533850, 0.01082677419508772804, 0.01181057656098392222, 0.01279437892688011814, 0.01377818129277631233, 0.01476198365867250825, 0.01525388484162060534, 0.01574578602456870244 ),
 .UNSPECIFIED. ) ;
#10681=EDGE_LOOP ( 'NONE', ( #20783, #18719, #6755, #14065, #19958, #20700, #17046 ) ) ;
#10701=VERTEX_POINT ( 'NONE', #19578 ) ;
#10704=DIRECTION ( 'NONE',  ( 0.000000000000000000, -1.000000000000000000, 0.000000000000000000 ) ) ;
#10712=VECTOR ( 'NONE', #17445, 1000.000000000000000 ) ;
#10763=ADVANCED_FACE ( 'NONE', ( #13746 ), #8536, .T. ) ;
#10790=ADVANCED_FACE ( 'NONE', ( #15055 ), #346, .F. ) ;
#10791=EDGE_LOOP ( 'NONE', ( #6963, #3249, #13535, #18158 ) ) ;
#10862=EDGE_CURVE ( 'NONE', #10281, #9782, #2810, .T. ) ;
#10872=ORIENTED_EDGE ( 'NONE', *, *, #3922, .T. ) ;
#10914=FACE_OUTER_BOUND ( 'NONE', #14625, .T. ) ;
#10962=VECTOR ( 'NONE', #18653, 1000.000000000000000 ) ;
#10969=CARTESIAN_POINT ( 'NONE',  ( -28.68588794268869435, 188.9102039777116602, 0.000000000000000000 ) ) ;
#11032=CARTESIAN_POINT ( 'NONE',  ( -11.06088464903280233, 326.0737056351150613, 5.773301668816269938 ) ) ;
#11054=CARTESIAN_POINT ( 'NONE',  ( -46.31968306282883674, 135.1716627696692683, 33.59072564020503648 ) ) ;
#11058=CARTESIAN_POINT ( 'NONE',  ( -41.83569717483972994, 213.9102039777116602, 24.99999999999998579 ) ) ;
#11087=DIRECTION ( 'NONE',  ( -1.191790137725560488E-16, 1.000000000000000000, -0.000000000000000000 ) ) ;
#11144=EDGE_CURVE ( 'NONE', #13614, #13852, #18037, .T. ) ;
#11228=CARTESIAN_POINT ( 'NONE',  ( -1.025382690249031503, 326.0737056351150613, -25.00000000000000000 ) ) ;
#11247=CARTESIAN_POINT ( 'NONE',  ( -43.60132883224871847, 209.8855831874335820, -1.619299207070721502 ) ) ;
#11250=EDGE_CURVE ( 'NONE', #21098, #2121, #19879, .T. ) ;
#11286=CARTESIAN_POINT ( 'NONE',  ( -11.06088464903280233, 326.0737056351150613, -5.773301668816269938 ) ) ;
#11394=DIRECTION ( 'NONE',  ( -1.191790137725560488E-16, 1.000000000000000000, -0.000000000000000000 ) ) ;
#11419=CIRCLE ( 'NONE', #19713, 5.000000000000001776 ) ;
#11422=CARTESIAN_POINT ( 'NONE',  ( -31.26501780185373391, 205.1437886375728965, 0.000000000000000000 ) ) ;
#11493=VECTOR ( 'NONE', #10382, 1000.000000000000000 ) ;
#11564=CARTESIAN_POINT ( 'NONE',  ( -43.68588794268869435, 200.1437886375728965, 2.403080215999224424E-15 ) ) ;
#11573=VERTEX_POINT ( 'NONE', #9043 ) ;
#11574=CARTESIAN_POINT ( 'NONE',  ( -42.82802356641965247, 205.4732429224858379, -5.000000000000002665 ) ) ;
#11613=LINE ( 'NONE', #4691, #613 ) ;
#11620=VECTOR ( 'NONE', #19493, 1000.000000000000000 ) ;
#11631=DIRECTION ( 'NONE',  ( -0.4627175328665442677, 0.000000000000000000, 0.8865057725575725689 ) ) ;
#11680=DIRECTION ( 'NONE',  ( 0.000000000000000000, 0.000000000000000000, 1.000000000000000000 ) ) ;
#11704=VERTEX_POINT ( 'NONE', #17802 ) ;
#11727=CARTESIAN_POINT ( 'NONE',  ( -43.31958977256851995, 208.9114094701607485, 3.303159798271270819 ) ) ;
#11730=LINE ( 'NONE', #5021, #16138 ) ;
#11743=ORIENTED_EDGE ( 'NONE', *, *, #6430, .F. ) ;
#11750=DIRECTION ( 'NONE',  ( -0.000000000000000000, 0.000000000000000000, 1.000000000000000000 ) ) ;
#11783=ORIENTED_EDGE ( 'NONE', *, *, #15335, .T. ) ;
#11833=CARTESIAN_POINT ( 'NONE',  ( -42.82802356641964536, 205.1437886375728965, 5.000000000000001776 ) ) ;
#11854=CARTESIAN_POINT ( 'NONE',  ( 0.000000000000000000, 326.0737056351150613, -25.00000000000000000 ) ) ;
#11860=CARTESIAN_POINT ( 'NONE',  ( -41.83569717483972994, 135.1716627696692683, 24.99999999999998934 ) ) ;
#11911=EDGE_LOOP ( 'NONE', ( #6726, #9395, #1288, #16508, #14777, #2269, #15005, #4973 ) ) ;
#11986=VECTOR ( 'NONE', #5675, 1000.000000000000000 ) ;
#12073=CARTESIAN_POINT ( 'NONE',  ( -42.82802356641964536, 205.1437886375728965, 5.000000000000001776 ) ) ;
#12108=EDGE_LOOP ( 'NONE', ( #897, #19848, #3983, #3679 ) ) ;
#12113=VECTOR ( 'NONE', #15912, 1000.000000000000000 ) ;
#12122=AXIS2_PLACEMENT_3D ( 'NONE', #18890, #15773, #962 ) ;
#12151=CARTESIAN_POINT ( 'NONE',  ( -43.47668584505344569, 200.8081422174835211, -2.511554223531087260 ) ) ;
#12161=MANIFOLD_SOLID_BREP ( 'Fillet4', #1762 ) ;
#12195=DIRECTION ( 'NONE',  ( 0.000000000000000000, 0.000000000000000000, 1.000000000000000000 ) ) ;
#12213=EDGE_CURVE ( 'NONE', #20916, #10281, #6835, .T. ) ;
#12224=ORIENTED_EDGE ( 'NONE', *, *, #13921, .F. ) ;
#12347=VERTEX_POINT ( 'NONE', #92 ) ;
#12404=ORIENTED_EDGE ( 'NONE', *, *, #2611, .F. ) ;
#12444=DIRECTION ( 'NONE',  ( -1.191790137725560488E-16, 1.000000000000000000, 0.000000000000000000 ) ) ;
#12531=CIRCLE ( 'NONE', #16676, 15.00000000000000355 ) ;
#12609=CARTESIAN_POINT ( 'NONE',  ( 18.55315245287936321, 130.1716627696692683, -25.00000000000000000 ) ) ;
#12630=EDGE_CURVE ( 'NONE', #13370, #1912, #2554, .T. ) ;
#12698=DIRECTION ( 'NONE',  ( 0.4627175328665442677, 0.000000000000000000, 0.8865057725575724579 ) ) ;
#12699=B_SPLINE_CURVE_WITH_KNOTS ( 'NONE', 3,
 ( #18629, #18954, #7058, #20693, #5866, #593, #10409, #14108, #10300, #13676, #9109, #2106, #2208, #12151, #7160, #13782, #20267, #18842, #16925, #811, #20483, #15515 ),
 .UNSPECIFIED., .F., .F.,
 ( 4, 2, 2, 2, 2, 2, 2, 2, 2, 2, 4 ),
 ( 0.02361608169583586866, 0.02460001686704667984, 0.02509198445265204552, 0.02558395203825741121, 0.02656788720946822238, 0.02755182238067903355, 0.02853575755188984125, 0.02951969272310065243, 0.03001166030870607362, 0.03050362789431149482, 0.03148756306552231987 ),
 .UNSPECIFIED. ) ;
#12711=CYLINDRICAL_SURFACE ( 'NONE', #13256, 5.000000000000001776 ) ;
#12729=ORIENTED_EDGE ( 'NONE', *, *, #15335, .F. ) ;
#12756=ORIENTED_EDGE ( 'NONE', *, *, #17290, .F. ) ;
#12766=CARTESIAN_POINT ( 'NONE',  ( -42.88695301665256920, 203.8419814082757568, 4.830353110044838694 ) ) ;
#12771=ORIENTED_EDGE ( 'NONE', *, *, #250, .F. ) ;
#12794=AXIS2_PLACEMENT_3D ( 'NONE', #808, #2419, #696 ) ;
#12820=MECHANICAL_DESIGN_GEOMETRIC_PRESENTATION_REPRESENTATION('',(#13177),#3488);
#12851=VECTOR ( 'NONE', #14813, 1000.000000000000000 ) ;
#12873=CARTESIAN_POINT ( 'NONE',  ( -42.82802356641964536, 205.1437886375728965, 5.000000000000001776 ) ) ;
#12875=PRODUCT_DEFINITION_SHAPE ( 'NONE', 'NONE',  #324 ) ;
#12878=EDGE_CURVE ( 'NONE', #7385, #14679, #10545, .T. ) ;
#12897=CARTESIAN_POINT ( 'NONE',  ( -46.31968306282883674, 213.9102039777116602, -33.59072564020502938 ) ) ;
#12924=DIRECTION ( 'NONE',  ( 0.4627175328665442677, 0.000000000000000000, -0.8865057725575724579 ) ) ;
#12925=CARTESIAN_POINT ( 'NONE',  ( 3.458603197740078627, 326.0737056351150613, 33.59072564020503648 ) ) ;
#13089=UNCERTAINTY_MEASURE_WITH_UNIT (LENGTH_MEASURE( 1.000000000000000082E-05 ), #13667, 'distance_accuracy_value', 'NONE');
#13140=DIRECTION ( 'NONE',  ( 0.4627175328665443232, 5.514621922230504147E-17, -0.8865057725575725689 ) ) ;
#13149=CYLINDRICAL_SURFACE ( 'NONE', #3066, 15.00000000000000355 ) ;
#13157=VERTEX_POINT ( 'NONE', #14433 ) ;
#13175=CARTESIAN_POINT ( 'NONE',  ( 0.000000000000000000, 135.1716627696692683, -33.59072564020503648 ) ) ;
#13177=STYLED_ITEM('',(#21421),#12161);
#13199=CARTESIAN_POINT ( 'NONE',  ( -43.04611869048239470, 202.6362012587621280, 4.338193544061892837 ) ) ;
#13256=AXIS2_PLACEMENT_3D ( 'NONE', #1045, #14241, #14350 ) ;
#13280=FACE_OUTER_BOUND ( 'NONE', #10358, .T. ) ;
#13315=DIRECTION ( 'NONE',  ( 1.000000000000000000, 0.000000000000000000, 0.000000000000000000 ) ) ;
#13336=CARTESIAN_POINT ( 'NONE',  ( 3.458603197740078627, 326.0737056351150613, -33.59072564020503648 ) ) ;
#13361=CARTESIAN_POINT ( 'NONE',  ( -43.52372910701232911, 209.6355236139544331, 2.220491386914096754 ) ) ;
#13370=VERTEX_POINT ( 'NONE', #4773 ) ;
#13386=PLANE ( 'NONE',  #19478 ) ;
#13424=DIRECTION ( 'NONE',  ( 0.000000000000000000, 0.000000000000000000, 1.000000000000000000 ) ) ;
#13446=ORIENTED_EDGE ( 'NONE', *, *, #14360, .T. ) ;
#13458=DIRECTION ( 'NONE',  ( -0.000000000000000000, 0.000000000000000000, 1.000000000000000000 ) ) ;
#13504=CIRCLE ( 'NONE', #1776, 15.00000000000000000 ) ;
#13505=ORIENTED_EDGE ( 'NONE', *, *, #5775, .T. ) ;
#13510=ORIENTED_EDGE ( 'NONE', *, *, #5782, .F. ) ;
#13520=EDGE_CURVE ( 'NONE', #661, #12347, #19594, .T. ) ;
#13535=ORIENTED_EDGE ( 'NONE', *, *, #13921, .T. ) ;
#13548=EDGE_CURVE ( 'NONE', #15417, #18006, #6497, .T. ) ;
#13600=CARTESIAN_POINT ( 'NONE',  ( 0.000000000000000000, 135.1716627696692683, 0.000000000000000000 ) ) ;
#13614=VERTEX_POINT ( 'NONE', #866 ) ;
#13661=LINE ( 'NONE', #13767, #15361 ) ;
#13667=( LENGTH_UNIT ( ) NAMED_UNIT ( * ) SI_UNIT ( .MILLI., .METRE. ) );
#13676=CARTESIAN_POINT ( 'NONE',  ( -43.15185836128297581, 202.0883771310975021, -3.971358459629989124 ) ) ;
#13733=APPLICATION_CONTEXT ( 'automotive_design' ) ;
#13746=FACE_OUTER_BOUND ( 'NONE', #1547, .T. ) ;
#13767=CARTESIAN_POINT ( 'NONE',  ( -11.06088464903280233, 135.1716627696692683, 5.773301668816269938 ) ) ;
#13782=CARTESIAN_POINT ( 'NONE',  ( -43.58160426315848213, 200.4655464737082013, -1.772246553899821997 ) ) ;
#13793=DIRECTION ( 'NONE',  ( -1.000000000000000000, -1.191790137725560488E-16, 0.000000000000000000 ) ) ;
#13807=DIRECTION ( 'NONE',  ( 0.000000000000000000, -1.000000000000000000, 0.000000000000000000 ) ) ;
#13820=VECTOR ( 'NONE', #13793, 1000.000000000000000 ) ;
#13822=DIRECTION ( 'NONE',  ( -1.000000000000000000, 0.000000000000000000, 0.000000000000000000 ) ) ;
#13852=VERTEX_POINT ( 'NONE', #19441 ) ;
#13916=LINE ( 'NONE', #5460, #11986 ) ;
#13921=EDGE_CURVE ( 'NONE', #9782, #12347, #6555, .T. ) ;
#13953=AXIS2_PLACEMENT_3D ( 'NONE', #11286, #3297, #12924 ) ;
#13957=LINE ( 'NONE', #3876, #10479 ) ;
#14065=ORIENTED_EDGE ( 'NONE', *, *, #17363, .T. ) ;
#14108=CARTESIAN_POINT ( 'NONE',  ( -42.99843930773591438, 202.9216059526226559, -4.490902998358449416 ) ) ;
#14114=ORIENTED_EDGE ( 'NONE', *, *, #13548, .T. ) ;
#14147=EDGE_LOOP ( 'NONE', ( #342, #19900, #12756, #3794 ) ) ;
#14188=DIRECTION ( 'NONE',  ( 0.000000000000000000, -1.000000000000000000, 0.000000000000000000 ) ) ;
#14195=( GEOMETRIC_REPRESENTATION_CONTEXT ( 3 ) GLOBAL_UNCERTAINTY_ASSIGNED_CONTEXT ( ( #8975 ) ) GLOBAL_UNIT_ASSIGNED_CONTEXT ( ( #15936, #5969, #19488 ) ) REPRESENTATION_CONTEXT ( 'NONE', 'WORKASPACE' ) );
#14236=EDGE_CURVE ( 'NONE', #3567, #18006, #8860, .T. ) ;
#14241=DIRECTION ( 'NONE',  ( -1.000000000000000000, -0.000000000000000000, -0.000000000000000000 ) ) ;
#14281=APPLICATION_CONTEXT ( 'automotive_design' ) ;
#14300=DIRECTION ( 'NONE',  ( 0.000000000000000000, -1.000000000000000000, 0.000000000000000000 ) ) ;
#14350=DIRECTION ( 'NONE',  ( 0.000000000000000000, 0.000000000000000000, 1.000000000000000000 ) ) ;
#14360=EDGE_CURVE ( 'NONE', #10701, #10452, #11730, .T. ) ;
#14370=EDGE_LOOP ( 'NONE', ( #12771, #1370, #873, #546 ) ) ;
#14421=DIRECTION ( 'NONE',  ( -1.000000000000000000, 0.000000000000000000, 0.000000000000000000 ) ) ;
#14432=CARTESIAN_POINT ( 'NONE',  ( -71.26501780185373036, 326.0737056351150613, -25.00000000000000355 ) ) ;
#14433=CARTESIAN_POINT ( 'NONE',  ( -71.26501780185373036, 205.1437886375728965, 5.000000000000001776 ) ) ;
#14505=CARTESIAN_POINT ( 'NONE',  ( -43.31820119254705759, 201.3816099220727835, 3.309203535948211261 ) ) ;
#14512=ORIENTED_EDGE ( 'NONE', *, *, #6445, .F. ) ;
#14550=PRODUCT_DEFINITION_FORMATION_WITH_SPECIFIED_SOURCE ( 'ANY', '', #9583, .NOT_KNOWN. ) ;
#14625=EDGE_LOOP ( 'NONE', ( #7350, #16589, #11743, #12404 ) ) ;
#14679=VERTEX_POINT ( 'NONE', #20486 ) ;
#14772=CARTESIAN_POINT ( 'NONE',  ( -43.20801099888741703, 208.4516271390267548, 3.763513762345671143 ) ) ;
#14777=ORIENTED_EDGE ( 'NONE', *, *, #12213, .T. ) ;
#14813=DIRECTION ( 'NONE',  ( 0.000000000000000000, -1.000000000000000000, 0.000000000000000000 ) ) ;
#14816=CARTESIAN_POINT ( 'NONE',  ( -71.26501780185373036, 205.1437886375728965, 0.000000000000000000 ) ) ;
#14837=CARTESIAN_POINT ( 'NONE',  ( -43.37409492154781532, 209.1153864038857932, -3.054836571872673101 ) ) ;
#14885=DIRECTION ( 'NONE',  ( -1.000000000000000000, -1.191790137725560488E-16, 0.000000000000000000 ) ) ;
#14909=CIRCLE ( 'NONE', #16618, 5.000000000000001776 ) ;
#14958=CARTESIAN_POINT ( 'NONE',  ( -13.68588794268869435, 188.9102039777116602, 1.836970198721029589E-15 ) ) ;
#15001=AXIS2_PLACEMENT_3D ( 'NONE', #19289, #2965, #12698 ) ;
#15005=ORIENTED_EDGE ( 'NONE', *, *, #11144, .F. ) ;
#15009=EDGE_CURVE ( 'NONE', #3359, #10360, #20290, .T. ) ;
#15016=DIRECTION ( 'NONE',  ( 0.4627175328665443232, 5.514621922230504147E-17, 0.8865057725575725689 ) ) ;
#15019=EDGE_CURVE ( 'NONE', #1471, #20916, #13916, .T. ) ;
#15052=ORIENTED_EDGE ( 'NONE', *, *, #10463, .F. ) ;
#15055=FACE_OUTER_BOUND ( 'NONE', #4177, .T. ) ;
#15097=CARTESIAN_POINT ( 'NONE',  ( -43.68588794268869435, 210.1437886375729533, 0.1639321870911856771 ) ) ;
#15335=EDGE_CURVE ( 'NONE', #4920, #6399, #11613, .T. ) ;
#15349=ORIENTED_EDGE ( 'NONE', *, *, #4926, .F. ) ;
#15353=EDGE_LOOP ( 'NONE', ( #21126, #5616 ) ) ;
#15361=VECTOR ( 'NONE', #5529, 1000.000000000000114 ) ;
#15374=DIRECTION ( 'NONE',  ( -1.000000000000000000, 0.000000000000000000, -0.000000000000000000 ) ) ;
#15417=VERTEX_POINT ( 'NONE', #4613 ) ;
#15515=CARTESIAN_POINT ( 'NONE',  ( -43.68588794268869435, 200.1437886375728965, 2.403080215999224424E-15 ) ) ;
#15543=EDGE_CURVE ( 'NONE', #10281, #13852, #4962, .T. ) ;
#15576=EDGE_CURVE ( 'NONE', #11573, #6728, #16120, .T. ) ;
#15585=VECTOR ( 'NONE', #854, 1000.000000000000000 ) ;
#15663=EDGE_CURVE ( 'NONE', #10452, #6038, #7080, .T. ) ;
#15708=EDGE_CURVE ( 'NONE', #1471, #74, #5464, .T. ) ;
#15731=LINE ( 'NONE', #4031, #3840 ) ;
#15773=DIRECTION ( 'NONE',  ( 1.000000000000000000, 0.000000000000000000, 0.000000000000000000 ) ) ;
#15799=DIRECTION ( 'NONE',  ( -0.4627175328665442677, 0.000000000000000000, -0.8865057725575725689 ) ) ;
#15860=FACE_OUTER_BOUND ( 'NONE', #17203, .T. ) ;
#15912=DIRECTION ( 'NONE',  ( 0.000000000000000000, 0.000000000000000000, 1.000000000000000000 ) ) ;
#15936=( LENGTH_UNIT ( ) NAMED_UNIT ( * ) SI_UNIT ( .MILLI., .METRE. ) );
#15997=LINE ( 'NONE', #2470, #1530 ) ;
#16011=ORIENTED_EDGE ( 'NONE', *, *, #3922, .F. ) ;
#16061=ADVANCED_FACE ( 'NONE', ( #21249 ), #16716, .F. ) ;
#16120=LINE ( 'NONE', #1846, #18563 ) ;
#16134=CARTESIAN_POINT ( 'NONE',  ( -43.68588794268869435, 210.1437886375728965, -2.161864096862809871E-19 ) ) ;
#16136=CARTESIAN_POINT ( 'NONE',  ( -46.31968306282883674, 213.9102039777116602, 33.59072564020503648 ) ) ;
#16138=VECTOR ( 'NONE', #14885, 1000.000000000000000 ) ;
#16179=CYLINDRICAL_SURFACE ( 'NONE', #9398, 15.00000000000000355 ) ;
#16181=EDGE_CURVE ( 'NONE', #10452, #7286, #6522, .T. ) ;
#16187=CARTESIAN_POINT ( 'NONE',  ( -28.68588794268869435, 188.9102039777116602, 0.000000000000000000 ) ) ;
#16231=CARTESIAN_POINT ( 'NONE',  ( -42.91921849944091605, 203.5275734399367025, 4.734433616062221795 ) ) ;
#16243=CARTESIAN_POINT ( 'NONE',  ( -43.67497163690817530, 210.1113231631600513, -0.6580207156766567644 ) ) ;
#16365=PRODUCT_DEFINITION_CONTEXT ( 'detailed design', #13733, 'design' ) ;
#16443=CARTESIAN_POINT ( 'NONE',  ( 18.55315245287936321, 326.0737056351150613, -25.00000000000000000 ) ) ;
#16452=CARTESIAN_POINT ( 'NONE',  ( 18.55315245287936321, 130.1716627696692683, 25.00000000000000000 ) ) ;
#16461=FACE_OUTER_BOUND ( 'NONE', #20729, .T. ) ;
#16508=ORIENTED_EDGE ( 'NONE', *, *, #15019, .T. ) ;
#16524=FACE_BOUND ( 'NONE', #2885, .T. ) ;
#16589=ORIENTED_EDGE ( 'NONE', *, *, #3542, .F. ) ;
#16602=PLANE ( 'NONE',  #13953 ) ;
#16618=AXIS2_PLACEMENT_3D ( 'NONE', #19001, #8938, #12195 ) ;
#16634=DIRECTION ( 'NONE',  ( -1.000000000000000000, -1.191790137725560488E-16, 0.000000000000000000 ) ) ;
#16676=AXIS2_PLACEMENT_3D ( 'NONE', #20570, #19264, #9197 ) ;
#16716=PLANE ( 'NONE',  #4387 ) ;
#16717=CARTESIAN_POINT ( 'NONE',  ( -43.66427838156418062, 210.0786766341574889, 0.8210443013742925178 ) ) ;
#16754=VERTEX_POINT ( 'NONE', #8006 ) ;
#16857=VECTOR ( 'NONE', #17734, 1000.000000000000000 ) ;
#16925=CARTESIAN_POINT ( 'NONE',  ( -43.64324723180579468, 200.2731091681331463, -1.141620385913092228 ) ) ;
#16939=ORIENTED_EDGE ( 'NONE', *, *, #12878, .F. ) ;
#16947=LINE ( 'NONE', #8709, #17707 ) ;
#16997=CARTESIAN_POINT ( 'NONE',  ( -46.31968306282883674, 135.1716627696692683, -33.59072564020502938 ) ) ;
#17042=EDGE_CURVE ( 'NONE', #7286, #18039, #17211, .T. ) ;
#17043=DIRECTION ( 'NONE',  ( 0.4627175328665443232, 5.514621922230504147E-17, -0.8865057725575725689 ) ) ;
#17046=ORIENTED_EDGE ( 'NONE', *, *, #14236, .T. ) ;
#17049=CIRCLE ( 'NONE', #7701, 25.00000000000000711 ) ;
#17179=CARTESIAN_POINT ( 'NONE',  ( -31.26501780185373391, 205.1437886375728965, 5.000000000000001776 ) ) ;
#17191=VECTOR ( 'NONE', #14300, 1000.000000000000000 ) ;
#17203=EDGE_LOOP ( 'NONE', ( #6783, #16011, #16939, #5848, #7201 ) ) ;
#17211=LINE ( 'NONE', #7774, #17191 ) ;
#17220=CARTESIAN_POINT ( 'NONE',  ( -71.26501780185373036, 326.0737056351150613, 25.00000000000000355 ) ) ;
#17290=EDGE_CURVE ( 'NONE', #10000, #21098, #4646, .T. ) ;
#17331=LINE ( 'NONE', #2514, #1410 ) ;
#17343=VECTOR ( 'NONE', #15016, 999.9999999999998863 ) ;
#17363=EDGE_CURVE ( 'NONE', #10360, #7385, #1300, .T. ) ;
#17445=DIRECTION ( 'NONE',  ( 0.000000000000000000, -1.000000000000000000, 0.000000000000000000 ) ) ;
#17463=PLANE ( 'NONE',  #333 ) ;
#17526=PLANE ( 'NONE',  #20413 ) ;
#17630=CARTESIAN_POINT ( 'NONE',  ( -28.68588794268869790, 213.9102039777116602, 0.000000000000000000 ) ) ;
#17666=ORIENTED_EDGE ( 'NONE', *, *, #777, .F. ) ;
#17667=PLANE ( 'NONE',  #15001 ) ;
#17701=CARTESIAN_POINT ( 'NONE',  ( -71.26501780185373036, 213.9102039777116602, -25.00000000000000355 ) ) ;
#17707=VECTOR ( 'NONE', #8274, 1000.000000000000000 ) ;
#17734=DIRECTION ( 'NONE',  ( 0.000000000000000000, -1.000000000000000000, 0.000000000000000000 ) ) ;
#17794=EDGE_LOOP ( 'NONE', ( #6537, #11783, #5629, #8151, #3314, #19025, #18112, #5507 ) ) ;
#17802=CARTESIAN_POINT ( 'NONE',  ( -1.025382690249029949, 135.1716627696692683, 25.00000000000000000 ) ) ;
#17836=CARTESIAN_POINT ( 'NONE',  ( 0.000000000000000000, 135.1716627696692683, 0.000000000000000000 ) ) ;
#17845=CARTESIAN_POINT ( 'NONE',  ( -43.52342829599624707, 209.6345393943126396, -2.222589281884806756 ) ) ;
#17895=ORIENTED_EDGE ( 'NONE', *, *, #5130, .T. ) ;
#17956=CARTESIAN_POINT ( 'NONE',  ( -71.26501780185373036, 135.1716627696692683, 25.00000000000000355 ) ) ;
#17999=CARTESIAN_POINT ( 'NONE',  ( -42.83990393396077678, 205.8064044967071879, 4.966739033517835189 ) ) ;
#18006=VERTEX_POINT ( 'NONE', #1713 ) ;
#18037=LINE ( 'NONE', #11228, #12851 ) ;
#18039=VERTEX_POINT ( 'NONE', #11860 ) ;
#18058=DIRECTION ( 'NONE',  ( -1.000000000000000000, -0.000000000000000000, -0.000000000000000000 ) ) ;
#18099=DIRECTION ( 'NONE',  ( -1.000000000000000000, 0.000000000000000000, -0.000000000000000000 ) ) ;
#18112=ORIENTED_EDGE ( 'NONE', *, *, #17042, .F. ) ;
#18152=CARTESIAN_POINT ( 'NONE',  ( -43.68588794268870146, 200.1437886375729249, 0.3330356950053358633 ) ) ;
#18158=ORIENTED_EDGE ( 'NONE', *, *, #38, .T. ) ;
#18196=PLANE ( 'NONE',  #20757 ) ;
#18201=LINE ( 'NONE', #1896, #9967 ) ;
#18265=VECTOR ( 'NONE', #6599, 1000.000000000000000 ) ;
#18320=CARTESIAN_POINT ( 'NONE',  ( -43.60140439023965797, 209.8858117899327169, 1.618481238659645882 ) ) ;
#18331=CARTESIAN_POINT ( 'NONE',  ( -11.06088464903280233, 135.1716627696692683, -5.773301668816269938 ) ) ;
#18368=VECTOR ( 'NONE', #15799, 1000.000000000000114 ) ;
#18416=PRODUCT_CONTEXT ( 'NONE', #14281, 'mechanical' ) ;
#18428=CARTESIAN_POINT ( 'NONE',  ( -42.91714575264039411, 206.7622684196151965, 4.742258924317273916 ) ) ;
#18488=CARTESIAN_POINT ( 'NONE',  ( 0.000000000000000000, 326.0737056351150613, 33.59072564020503648 ) ) ;
#18512=EDGE_CURVE ( 'NONE', #6728, #11704, #8870, .T. ) ;
#18551=DIRECTION ( 'NONE',  ( 0.000000000000000000, 0.000000000000000000, -1.000000000000000000 ) ) ;
#18563=VECTOR ( 'NONE', #3952, 1000.000000000000000 ) ;
#18629=CARTESIAN_POINT ( 'NONE',  ( -42.82802356641964536, 205.1437886375728965, -5.000000000000001776 ) ) ;
#18636=ORIENTED_EDGE ( 'NONE', *, *, #10463, .T. ) ;
#18653=DIRECTION ( 'NONE',  ( 0.000000000000000000, 0.000000000000000000, 1.000000000000000000 ) ) ;
#18719=ORIENTED_EDGE ( 'NONE', *, *, #8284, .F. ) ;
#18735=DIRECTION ( 'NONE',  ( -1.000000000000000000, 0.000000000000000000, -0.000000000000000000 ) ) ;
#18842=CARTESIAN_POINT ( 'NONE',  ( -43.63022347157595249, 200.3131325479158704, -1.300740588846951651 ) ) ;
#18890=CARTESIAN_POINT ( 'NONE',  ( 18.55315245287936321, 130.1716627696692683, 1.734723475976807094E-15 ) ) ;
#18954=CARTESIAN_POINT ( 'NONE',  ( -42.82802356641966668, 204.8142847187656059, -5.000000000000003553 ) ) ;
#18959=AXIS2_PLACEMENT_3D ( 'NONE', #275, #18735, #13458 ) ;
#19001=CARTESIAN_POINT ( 'NONE',  ( -71.26501780185373036, 205.1437886375728965, 0.000000000000000000 ) ) ;
#19025=ORIENTED_EDGE ( 'NONE', *, *, #7856, .T. ) ;
#19027=CARTESIAN_POINT ( 'NONE',  ( -22.62331590640576451, 135.1716627696692683, 11.80838889663595914 ) ) ;
#19264=DIRECTION ( 'NONE',  ( -1.191790137725560488E-16, 1.000000000000000000, 0.000000000000000000 ) ) ;
#19289=CARTESIAN_POINT ( 'NONE',  ( -22.62331590640576451, 326.0737056351150613, 11.80838889663595914 ) ) ;
#19309=DIRECTION ( 'NONE',  ( -1.191790137725560488E-16, 1.000000000000000000, 0.000000000000000000 ) ) ;
#19357=LINE ( 'NONE', #9297, #12113 ) ;
#19364=ADVANCED_FACE ( 'NONE', ( #8918 ), #2235, .T. ) ;
#19365=ORIENTED_EDGE ( 'NONE', *, *, #9348, .F. ) ;
#19441=CARTESIAN_POINT ( 'NONE',  ( -1.025382690249031503, 135.1716627696692683, -25.00000000000000000 ) ) ;
#19478=AXIS2_PLACEMENT_3D ( 'NONE', #8389, #19974, #11750 ) ;
#19488=( NAMED_UNIT ( * ) SI_UNIT ( $, .STERADIAN. ) SOLID_ANGLE_UNIT ( ) );
#19493=DIRECTION ( 'NONE',  ( -1.191790137725560488E-16, 1.000000000000000000, -0.000000000000000000 ) ) ;
#19499=ORIENTED_EDGE ( 'NONE', *, *, #12213, .F. ) ;
#19524=FACE_OUTER_BOUND ( 'NONE', #6903, .T. ) ;
#19576=CARTESIAN_POINT ( 'NONE',  ( -42.99872675744467188, 207.3681867157733905, -4.490020761129742688 ) ) ;
#19578=CARTESIAN_POINT ( 'NONE',  ( 3.458603197740082180, 213.9102039777116602, 33.59072564020503648 ) ) ;
#19594=LINE ( 'NONE', #13336, #3332 ) ;
#19659=ADVANCED_FACE ( 'NONE', ( #15860 ), #12711, .F. ) ;
#19689=PLANE ( 'NONE',  #5135 ) ;
#19712=ADVANCED_FACE ( 'NONE', ( #2978 ), #16602, .T. ) ;
#19713=AXIS2_PLACEMENT_3D ( 'NONE', #14816, #14421, #4449 ) ;
#19848=ORIENTED_EDGE ( 'NONE', *, *, #16181, .T. ) ;
#19879=LINE ( 'NONE', #10340, #21139 ) ;
#19900=ORIENTED_EDGE ( 'NONE', *, *, #1284, .T. ) ;
#19958=ORIENTED_EDGE ( 'NONE', *, *, #12878, .T. ) ;
#19974=DIRECTION ( 'NONE',  ( -1.000000000000000000, 0.000000000000000000, -0.000000000000000000 ) ) ;
#20011=EDGE_LOOP ( 'NONE', ( #15349, #6018, #4342, #8828, #9681 ) ) ;
#20042=CARTESIAN_POINT ( 'NONE',  ( -41.83569717483972994, 326.0737056351150613, -24.99999999999998934 ) ) ;
#20118=CARTESIAN_POINT ( 'NONE',  ( -71.26501780185373036, 130.1716627696692683, 1.734723475976807094E-15 ) ) ;
#20147=ORIENTED_EDGE ( 'NONE', *, *, #15708, .F. ) ;
#20187=PLANE ( 'NONE',  #4245 ) ;
#20221=ORIENTED_EDGE ( 'NONE', *, *, #11250, .F. ) ;
#20256=( NAMED_UNIT ( * ) SI_UNIT ( $, .STERADIAN. ) SOLID_ANGLE_UNIT ( ) );
#20267=CARTESIAN_POINT ( 'NONE',  ( -43.59942232657300565, 200.4092789822994121, -1.616039188923340308 ) ) ;
#20279=CARTESIAN_POINT ( 'NONE',  ( 1.336753550880579347E-14, 213.9102039777116602, -33.59072564020503648 ) ) ;
#20290=LINE ( 'NONE', #7180, #9218 ) ;
#20325=VECTOR ( 'NONE', #9735, 1000.000000000000000 ) ;
#20332=CARTESIAN_POINT ( 'NONE',  ( -71.26501780185373036, 130.1716627696692683, 1.734723475976807094E-15 ) ) ;
#20370=CARTESIAN_POINT ( 'NONE',  ( -71.26501780185373036, 130.1716627696692683, 25.00000000000000355 ) ) ;
#20413=AXIS2_PLACEMENT_3D ( 'NONE', #17836, #14188, #20780 ) ;
#20478=CARTESIAN_POINT ( 'NONE',  ( -43.68588794268869435, 188.9102039777116602, 0.000000000000000000 ) ) ;
#20483=CARTESIAN_POINT ( 'NONE',  ( -43.68588794268868725, 200.1437886375728397, -0.3328713742805504139 ) ) ;
#20486=CARTESIAN_POINT ( 'NONE',  ( -43.68588794268869435, 210.1437886375728965, -2.161864096862809871E-19 ) ) ;
#20519=ORIENTED_EDGE ( 'NONE', *, *, #4926, .T. ) ;
#20538=ADVANCED_FACE ( 'NONE', ( #9901 ), #20187, .T. ) ;
#20547=ORIENTED_EDGE ( 'NONE', *, *, #15576, .F. ) ;
#20570=CARTESIAN_POINT ( 'NONE',  ( -28.68588794268869435, 188.9102039777116602, 0.000000000000000000 ) ) ;
#20586=EDGE_CURVE ( 'NONE', #74, #7286, #16947, .T. ) ;
#20693=CARTESIAN_POINT ( 'NONE',  ( -42.87301415892787304, 204.0033847496196699, -4.870997244581529273 ) ) ;
#20700=ORIENTED_EDGE ( 'NONE', *, *, #9348, .T. ) ;
#20729=EDGE_LOOP ( 'NONE', ( #9512, #7461, #8047, #5033, #20547, #13510, #262, #5215, #18636, #5265, #3982, #6967 ) ) ;
#20757=AXIS2_PLACEMENT_3D ( 'NONE', #9861, #1670, #6512 ) ;
#20780=DIRECTION ( 'NONE',  ( 0.000000000000000000, -0.000000000000000000, -1.000000000000000000 ) ) ;
#20783=ORIENTED_EDGE ( 'NONE', *, *, #13548, .F. ) ;
#20836=CARTESIAN_POINT ( 'NONE',  ( -28.68588794268869790, 213.9102039777116602, 0.000000000000000000 ) ) ;
#20904=SHAPE_REPRESENTATION_RELATIONSHIP ( 'NONE' , 'NONE' ,  #7793, #7899 ) ;
#20916=VERTEX_POINT ( 'NONE', #5677 ) ;
#21098=VERTEX_POINT ( 'NONE', #12609 ) ;
#21099=CARTESIAN_POINT ( 'NONE',  ( -43.68588794268869435, 210.1437886375729249, -0.3278592396120701968 ) ) ;
#21108=EDGE_CURVE ( 'NONE', #10701, #16754, #4489, .T. ) ;
#21126=ORIENTED_EDGE ( 'NONE', *, *, #14236, .F. ) ;
#21139=VECTOR ( 'NONE', #13822, 1000.000000000000000 ) ;
#21157=ORIENTED_EDGE ( 'NONE', *, *, #13520, .T. ) ;
#21170=CARTESIAN_POINT ( 'NONE',  ( -11.06088464903279878, 213.9102039777116602, 5.773301668816275267 ) ) ;
#21249=FACE_OUTER_BOUND ( 'NONE', #17794, .T. ) ;
#21282=ORIENTED_EDGE ( 'NONE', *, *, #5077, .F. ) ;
#21295=VECTOR ( 'NONE', #10127, 1000.000000000000000 ) ;
#21296=CARTESIAN_POINT ( 'NONE',  ( -42.82802356641963826, 204.8148611821455916, 5.000000000000001776 ) ) ;
#21415=COLOUR_RGB('Light Blue',0.38,0.62,0.78);
#21416=FILL_AREA_STYLE_COLOUR('',#21415);
#21417=FILL_AREA_STYLE('',(#21416));
#21418=SURFACE_STYLE_FILL_AREA(#21417);
#21419=SURFACE_SIDE_STYLE('',(#21418));
#21420=SURFACE_STYLE_USAGE(.BOTH.,#21419);
#21421=PRESENTATION_STYLE_ASSIGNMENT((#21420));
ENDSEC;
END-ISO-10303-21;
